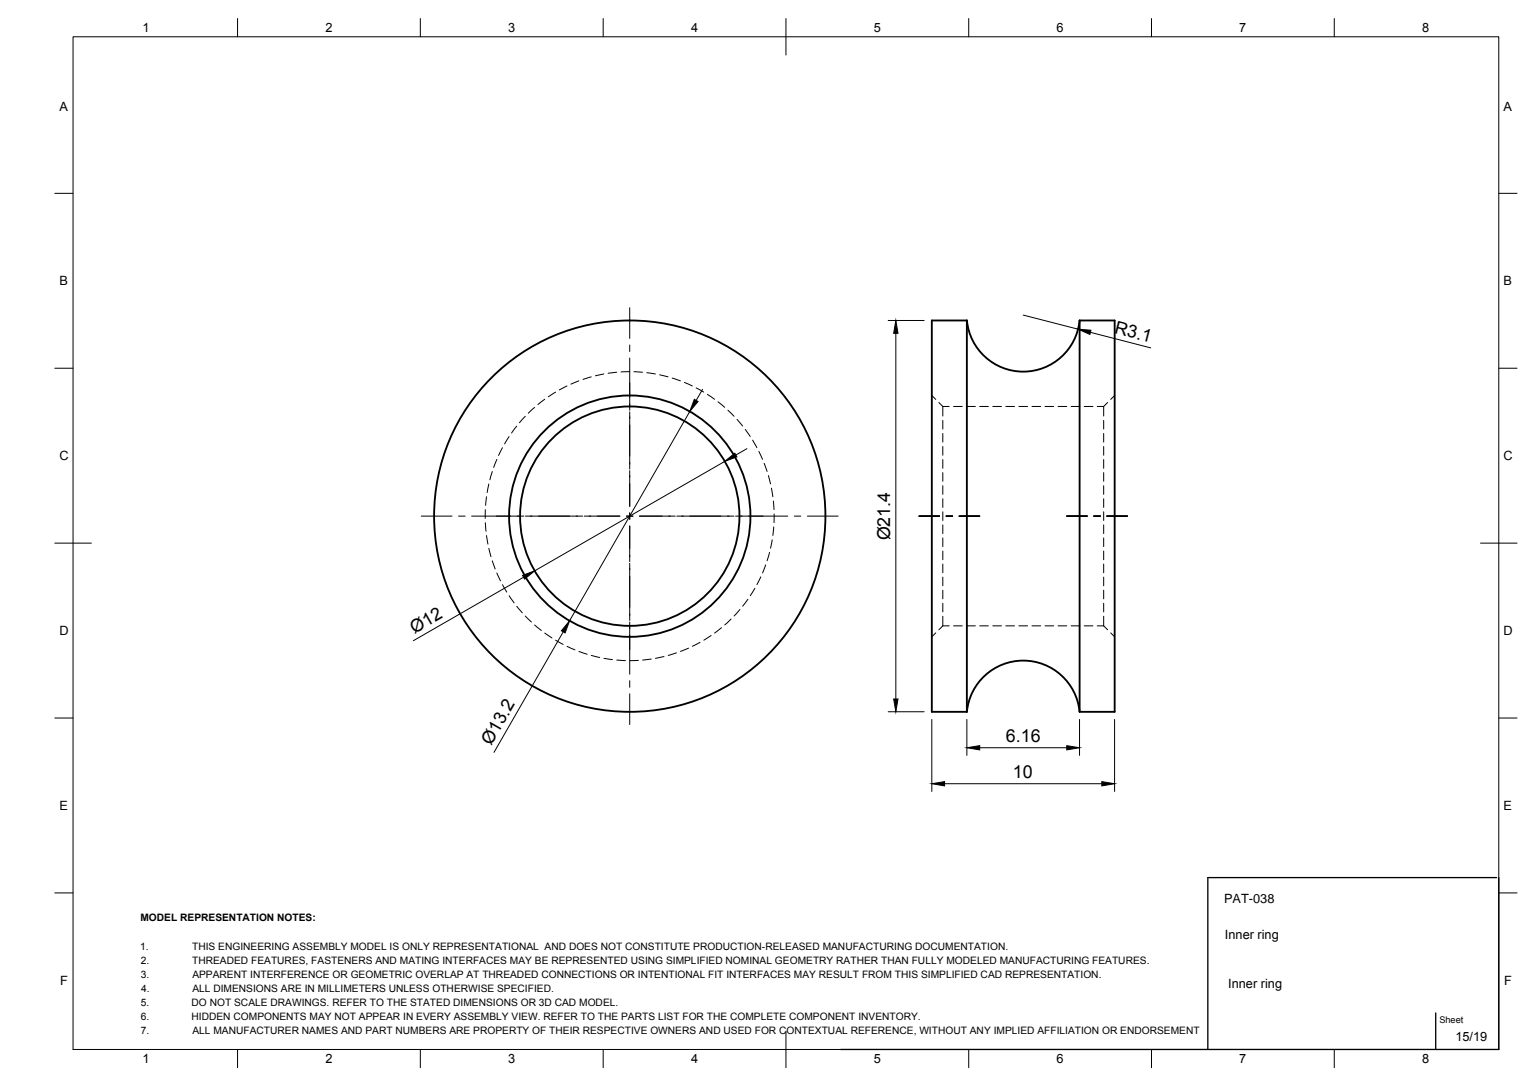
ISO-10303-21;
HEADER;
/* Generated by software containing ST-Developer
 * from STEP Tools, Inc. (www.steptools.com) 
 */

FILE_DESCRIPTION(
/* description */ ('Fork-mounted skate wheel'),
/* implementation_level */ '2;1');

FILE_NAME(
/* name */ 'Inner ring.step',
/* time_stamp */ '2026-10-29T16:11:26-07:00',
/* author */ (''),
/* organization */ (''),
/* preprocessor_version */ 'ST-DEVELOPER v20.2',
/* originating_system */ 'Autodesk Translation Framework v15.17.0.0',
/* authorisation */ '');

FILE_SCHEMA (('AUTOMOTIVE_DESIGN { 1 0 10303 214 3 1 1 }'));
ENDSEC;

DATA;
#10=MECHANICAL_DESIGN_GEOMETRIC_PRESENTATION_REPRESENTATION('',(#152),#3688);
#39=TOROIDAL_SURFACE('',#2079,1.1,0.309556);
#116=CONICAL_SURFACE('',#2090,0.63,0.785398163397448);
#117=CONICAL_SURFACE('',#2097,0.63,0.785398163397448);
#128=SHAPE_REPRESENTATION_RELATIONSHIP('SRR','None',#3753,#140);
#140=ADVANCED_BREP_SHAPE_REPRESENTATION('',(#170),#3682);
#152=STYLED_ITEM('',(#3896),#170);
#170=MANIFOLD_SOLID_BREP('Body1',#1814);
#208=FACE_BOUND('',#480,.T.);
#209=FACE_BOUND('',#483,.T.);
#258=PLANE('',#2092);
#259=PLANE('',#2095);
#337=FACE_OUTER_BOUND('',#475,.T.);
#338=FACE_OUTER_BOUND('',#476,.T.);
#339=FACE_OUTER_BOUND('',#477,.T.);
#340=FACE_OUTER_BOUND('',#478,.T.);
#341=FACE_OUTER_BOUND('',#479,.T.);
#342=FACE_OUTER_BOUND('',#481,.T.);
#343=FACE_OUTER_BOUND('',#482,.T.);
#344=FACE_OUTER_BOUND('',#484,.T.);
#475=EDGE_LOOP('',(#1451,#1452,#1453,#1454,#1455,#1456));
#476=EDGE_LOOP('',(#1457,#1458,#1459,#1460,#1461));
#477=EDGE_LOOP('',(#1462,#1463,#1464,#1465));
#478=EDGE_LOOP('',(#1466,#1467,#1468,#1469));
#479=EDGE_LOOP('',(#1470));
#480=EDGE_LOOP('',(#1471));
#481=EDGE_LOOP('',(#1472,#1473,#1474,#1475,#1476));
#482=EDGE_LOOP('',(#1477));
#483=EDGE_LOOP('',(#1478));
#484=EDGE_LOOP('',(#1479,#1480,#1481,#1482));
#614=LINE('',#3121,#708);
#615=LINE('',#3127,#709);
#616=LINE('',#3131,#710);
#617=LINE('',#3137,#711);
#618=LINE('',#3142,#712);
#708=VECTOR('',#2549,1.070235);
#709=VECTOR('',#2556,0.6);
#710=VECTOR('',#2561,0.63);
#711=VECTOR('',#2570,1.070235);
#712=VECTOR('',#2577,0.63);
#767=CIRCLE('',#2080,1.070235);
#768=CIRCLE('',#2081,1.070235);
#769=CIRCLE('',#2082,0.309556);
#770=CIRCLE('',#2083,1.070235);
#771=CIRCLE('',#2084,1.070235);
#772=CIRCLE('',#2086,1.070235);
#773=CIRCLE('',#2088,0.6);
#774=CIRCLE('',#2089,0.6);
#775=CIRCLE('',#2091,0.66);
#776=CIRCLE('',#2094,1.070235);
#777=CIRCLE('',#2096,0.66);
#917=VERTEX_POINT('',#3110);
#918=VERTEX_POINT('',#3111);
#919=VERTEX_POINT('',#3114);
#920=VERTEX_POINT('',#3116);
#921=VERTEX_POINT('',#3120);
#922=VERTEX_POINT('',#3124);
#923=VERTEX_POINT('',#3126);
#924=VERTEX_POINT('',#3130);
#925=VERTEX_POINT('',#3135);
#926=VERTEX_POINT('',#3139);
#1112=EDGE_CURVE('',#917,#918,#767,.T.);
#1113=EDGE_CURVE('',#918,#917,#768,.T.);
#1114=EDGE_CURVE('',#918,#919,#769,.T.);
#1115=EDGE_CURVE('',#920,#919,#770,.T.);
#1116=EDGE_CURVE('',#919,#920,#771,.T.);
#1117=EDGE_CURVE('',#920,#921,#614,.T.);
#1118=EDGE_CURVE('',#921,#921,#772,.T.);
#1119=EDGE_CURVE('',#922,#922,#773,.T.);
#1120=EDGE_CURVE('',#922,#923,#615,.T.);
#1121=EDGE_CURVE('',#923,#923,#774,.T.);
#1122=EDGE_CURVE('',#923,#924,#616,.T.);
#1123=EDGE_CURVE('',#924,#924,#775,.T.);
#1124=EDGE_CURVE('',#925,#925,#776,.T.);
#1125=EDGE_CURVE('',#925,#917,#617,.T.);
#1126=EDGE_CURVE('',#926,#926,#777,.T.);
#1127=EDGE_CURVE('',#926,#922,#618,.T.);
#1451=ORIENTED_EDGE('',*,*,#1112,.F.);
#1452=ORIENTED_EDGE('',*,*,#1113,.F.);
#1453=ORIENTED_EDGE('',*,*,#1114,.T.);
#1454=ORIENTED_EDGE('',*,*,#1115,.F.);
#1455=ORIENTED_EDGE('',*,*,#1116,.F.);
#1456=ORIENTED_EDGE('',*,*,#1114,.F.);
#1457=ORIENTED_EDGE('',*,*,#1115,.T.);
#1458=ORIENTED_EDGE('',*,*,#1116,.T.);
#1459=ORIENTED_EDGE('',*,*,#1117,.T.);
#1460=ORIENTED_EDGE('',*,*,#1118,.T.);
#1461=ORIENTED_EDGE('',*,*,#1117,.F.);
#1462=ORIENTED_EDGE('',*,*,#1119,.T.);
#1463=ORIENTED_EDGE('',*,*,#1120,.T.);
#1464=ORIENTED_EDGE('',*,*,#1121,.F.);
#1465=ORIENTED_EDGE('',*,*,#1120,.F.);
#1466=ORIENTED_EDGE('',*,*,#1121,.T.);
#1467=ORIENTED_EDGE('',*,*,#1122,.T.);
#1468=ORIENTED_EDGE('',*,*,#1123,.F.);
#1469=ORIENTED_EDGE('',*,*,#1122,.F.);
#1470=ORIENTED_EDGE('',*,*,#1118,.F.);
#1471=ORIENTED_EDGE('',*,*,#1123,.T.);
#1472=ORIENTED_EDGE('',*,*,#1124,.F.);
#1473=ORIENTED_EDGE('',*,*,#1125,.T.);
#1474=ORIENTED_EDGE('',*,*,#1112,.T.);
#1475=ORIENTED_EDGE('',*,*,#1113,.T.);
#1476=ORIENTED_EDGE('',*,*,#1125,.F.);
#1477=ORIENTED_EDGE('',*,*,#1124,.T.);
#1478=ORIENTED_EDGE('',*,*,#1126,.F.);
#1479=ORIENTED_EDGE('',*,*,#1126,.T.);
#1480=ORIENTED_EDGE('',*,*,#1127,.T.);
#1481=ORIENTED_EDGE('',*,*,#1119,.F.);
#1482=ORIENTED_EDGE('',*,*,#1127,.F.);
#1680=CYLINDRICAL_SURFACE('',#2085,1.070235);
#1681=CYLINDRICAL_SURFACE('',#2087,0.6);
#1682=CYLINDRICAL_SURFACE('',#2093,1.070235);
#1755=ADVANCED_FACE('',(#337),#39,.F.);
#1756=ADVANCED_FACE('',(#338),#1680,.T.);
#1757=ADVANCED_FACE('',(#339),#1681,.F.);
#1758=ADVANCED_FACE('',(#340),#116,.F.);
#1759=ADVANCED_FACE('',(#341,#208),#258,.T.);
#1760=ADVANCED_FACE('',(#342),#1682,.T.);
#1761=ADVANCED_FACE('',(#343,#209),#259,.T.);
#1762=ADVANCED_FACE('',(#344),#117,.F.);
#1814=CLOSED_SHELL('',(#1755,#1756,#1757,#1758,#1759,#1760,#1761,#1762));
#2078=AXIS2_PLACEMENT_3D('',#3108,#2533,#2534);
#2079=AXIS2_PLACEMENT_3D('',#3109,#2535,#2536);
#2080=AXIS2_PLACEMENT_3D('',#3112,#2537,#2538);
#2081=AXIS2_PLACEMENT_3D('',#3113,#2539,#2540);
#2082=AXIS2_PLACEMENT_3D('',#3115,#2541,#2542);
#2083=AXIS2_PLACEMENT_3D('',#3117,#2543,#2544);
#2084=AXIS2_PLACEMENT_3D('',#3118,#2545,#2546);
#2085=AXIS2_PLACEMENT_3D('',#3119,#2547,#2548);
#2086=AXIS2_PLACEMENT_3D('',#3122,#2550,#2551);
#2087=AXIS2_PLACEMENT_3D('',#3123,#2552,#2553);
#2088=AXIS2_PLACEMENT_3D('',#3125,#2554,#2555);
#2089=AXIS2_PLACEMENT_3D('',#3128,#2557,#2558);
#2090=AXIS2_PLACEMENT_3D('',#3129,#2559,#2560);
#2091=AXIS2_PLACEMENT_3D('',#3132,#2562,#2563);
#2092=AXIS2_PLACEMENT_3D('',#3133,#2564,#2565);
#2093=AXIS2_PLACEMENT_3D('',#3134,#2566,#2567);
#2094=AXIS2_PLACEMENT_3D('',#3136,#2568,#2569);
#2095=AXIS2_PLACEMENT_3D('',#3138,#2571,#2572);
#2096=AXIS2_PLACEMENT_3D('',#3140,#2573,#2574);
#2097=AXIS2_PLACEMENT_3D('',#3141,#2575,#2576);
#2533=DIRECTION('axis',(0.,0.,1.));
#2534=DIRECTION('refdir',(1.,0.,0.));
#2535=DIRECTION('center_axis',(0.,-1.,0.));
#2536=DIRECTION('ref_axis',(0.,0.,-1.));
#2537=DIRECTION('center_axis',(0.,-1.,0.));
#2538=DIRECTION('ref_axis',(1.,0.,0.));
#2539=DIRECTION('center_axis',(0.,-1.,0.));
#2540=DIRECTION('ref_axis',(1.,0.,0.));
#2541=DIRECTION('center_axis',(1.,0.,1.22464679914735E-16));
#2542=DIRECTION('ref_axis',(-1.22464679914735E-16,0.,1.));
#2543=DIRECTION('center_axis',(0.,1.,0.));
#2544=DIRECTION('ref_axis',(1.,0.,0.));
#2545=DIRECTION('center_axis',(0.,1.,0.));
#2546=DIRECTION('ref_axis',(1.,0.,0.));
#2547=DIRECTION('center_axis',(0.,-1.,0.));
#2548=DIRECTION('ref_axis',(1.,0.,0.));
#2549=DIRECTION('',(0.,1.,0.));
#2550=DIRECTION('center_axis',(0.,-1.,0.));
#2551=DIRECTION('ref_axis',(1.,0.,0.));
#2552=DIRECTION('center_axis',(0.,-1.,0.));
#2553=DIRECTION('ref_axis',(1.,0.,0.));
#2554=DIRECTION('center_axis',(0.,-1.,0.));
#2555=DIRECTION('ref_axis',(1.,0.,0.));
#2556=DIRECTION('',(0.,1.,0.));
#2557=DIRECTION('center_axis',(0.,-1.,0.));
#2558=DIRECTION('ref_axis',(1.,0.,0.));
#2559=DIRECTION('center_axis',(0.,1.,0.));
#2560=DIRECTION('ref_axis',(1.,0.,0.));
#2561=DIRECTION('',(-0.707106781186548,0.707106781186547,-8.65956056235493E-17));
#2562=DIRECTION('center_axis',(0.,-1.,0.));
#2563=DIRECTION('ref_axis',(1.,0.,0.));
#2564=DIRECTION('center_axis',(0.,1.,0.));
#2565=DIRECTION('ref_axis',(0.,0.,1.));
#2566=DIRECTION('center_axis',(0.,-1.,0.));
#2567=DIRECTION('ref_axis',(1.,0.,0.));
#2568=DIRECTION('center_axis',(0.,-1.,0.));
#2569=DIRECTION('ref_axis',(1.,0.,0.));
#2570=DIRECTION('',(0.,1.,0.));
#2571=DIRECTION('center_axis',(0.,-1.,0.));
#2572=DIRECTION('ref_axis',(0.,0.,-1.));
#2573=DIRECTION('center_axis',(0.,-1.,0.));
#2574=DIRECTION('ref_axis',(1.,0.,0.));
#2575=DIRECTION('center_axis',(0.,-1.,0.));
#2576=DIRECTION('ref_axis',(1.,0.,0.));
#2577=DIRECTION('',(0.707106781186548,0.707106781186547,8.65956056235493E-17));
#3108=CARTESIAN_POINT('',(0.,0.,0.));
#3109=CARTESIAN_POINT('Origin',(0.,0.,0.));
#3110=CARTESIAN_POINT('',(-1.070235,-0.308121667383195,-1.31065986708547E-16));
#3111=CARTESIAN_POINT('',(-1.31065986708547E-16,-0.308121667383195,1.070235));
#3112=CARTESIAN_POINT('Origin',(0.,-0.308121667383195,0.));
#3113=CARTESIAN_POINT('Origin',(0.,-0.308121667383195,0.));
#3114=CARTESIAN_POINT('',(-1.31065986708547E-16,0.308121667383195,1.070235));
#3115=CARTESIAN_POINT('Origin',(-1.34711147906209E-16,0.,1.1));
#3116=CARTESIAN_POINT('',(-1.070235,0.308121667383195,1.31065986708547E-16));
#3117=CARTESIAN_POINT('Origin',(0.,0.308121667383195,0.));
#3118=CARTESIAN_POINT('Origin',(0.,0.308121667383195,0.));
#3119=CARTESIAN_POINT('Origin',(0.,0.,0.));
#3120=CARTESIAN_POINT('',(-1.070235,0.5,-1.31065986708547E-16));
#3121=CARTESIAN_POINT('',(-1.070235,0.,-1.31065986708547E-16));
#3122=CARTESIAN_POINT('Origin',(0.,0.5,0.));
#3123=CARTESIAN_POINT('Origin',(0.,0.,0.));
#3124=CARTESIAN_POINT('',(-0.6,-0.44,-7.34788079488412E-17));
#3125=CARTESIAN_POINT('Origin',(0.,-0.44,0.));
#3126=CARTESIAN_POINT('',(-0.6,0.44,-7.34788079488412E-17));
#3127=CARTESIAN_POINT('',(-0.6,0.,-7.34788079488412E-17));
#3128=CARTESIAN_POINT('Origin',(0.,0.44,0.));
#3129=CARTESIAN_POINT('Origin',(0.,0.47,0.));
#3130=CARTESIAN_POINT('',(-0.66,0.5,-8.08266887437253E-17));
#3131=CARTESIAN_POINT('',(-0.63,0.47,-7.71527483462832E-17));
#3132=CARTESIAN_POINT('Origin',(0.,0.5,0.));
#3133=CARTESIAN_POINT('Origin',(1.070235,0.5,0.));
#3134=CARTESIAN_POINT('Origin',(0.,0.,0.));
#3135=CARTESIAN_POINT('',(-1.070235,-0.5,-1.31065986708547E-16));
#3136=CARTESIAN_POINT('Origin',(0.,-0.5,0.));
#3137=CARTESIAN_POINT('',(-1.070235,0.,-1.31065986708547E-16));
#3138=CARTESIAN_POINT('Origin',(0.66,-0.5,0.));
#3139=CARTESIAN_POINT('',(-0.66,-0.5,-8.08266887437253E-17));
#3140=CARTESIAN_POINT('Origin',(0.,-0.5,0.));
#3141=CARTESIAN_POINT('Origin',(0.,-0.47,0.));
#3142=CARTESIAN_POINT('',(-0.63,-0.47,-7.71527483462832E-17));
#3665=UNCERTAINTY_MEASURE_WITH_UNIT(LENGTH_MEASURE(0.001),#3689,
'DISTANCE_ACCURACY_VALUE',
'Maximum model space distance between geometric entities at asserted c
onnectivities');
#3671=UNCERTAINTY_MEASURE_WITH_UNIT(LENGTH_MEASURE(0.001),#3689,
'DISTANCE_ACCURACY_VALUE',
'Maximum model space distance between geometric entities at asserted c
onnectivities');
#3682=(
GEOMETRIC_REPRESENTATION_CONTEXT(3)
GLOBAL_UNCERTAINTY_ASSIGNED_CONTEXT((#3665))
GLOBAL_UNIT_ASSIGNED_CONTEXT((#3689,#3691,#3692))
REPRESENTATION_CONTEXT('','3D')
);
#3688=(
GEOMETRIC_REPRESENTATION_CONTEXT(3)
GLOBAL_UNCERTAINTY_ASSIGNED_CONTEXT((#3671))
GLOBAL_UNIT_ASSIGNED_CONTEXT((#3689,#3691,#3692))
REPRESENTATION_CONTEXT('','3D')
);
#3689=(
LENGTH_UNIT()
NAMED_UNIT(*)
SI_UNIT(.CENTI.,.METRE.)
);
#3691=(
NAMED_UNIT(*)
PLANE_ANGLE_UNIT()
SI_UNIT($,.RADIAN.)
);
#3692=(
NAMED_UNIT(*)
SI_UNIT($,.STERADIAN.)
SOLID_ANGLE_UNIT()
);
#3703=SHAPE_DEFINITION_REPRESENTATION(#3725,#3753);
#3725=PRODUCT_DEFINITION_SHAPE('',$,#3770);
#3753=SHAPE_REPRESENTATION('',(#2078),#3682);
#3759=PRODUCT_DEFINITION_CONTEXT('part definition',#3809,'design');
#3770=PRODUCT_DEFINITION('Inner ring','Inner ring',#3786,#3759);
#3786=PRODUCT_DEFINITION_FORMATION('',$,#3821);
#3809=APPLICATION_CONTEXT(
'Core Data for Automotive Mechanical Design Process');
#3810=PRODUCT_CONTEXT('part definition',#3809,'mechanical');
#3821=PRODUCT('Inner ring','Inner ring','Inner ring',(#3810));
#3890=COLOUR_RGB('Grey',0.48,0.52,0.57);
#3891=FILL_AREA_STYLE_COLOUR('',#3890);
#3892=FILL_AREA_STYLE('',(#3891));
#3893=SURFACE_STYLE_FILL_AREA(#3892);
#3894=SURFACE_SIDE_STYLE('',(#3893));
#3895=SURFACE_STYLE_USAGE(.BOTH.,#3894);
#3896=PRESENTATION_STYLE_ASSIGNMENT((#3895));
ENDSEC;
END-ISO-10303-21;
